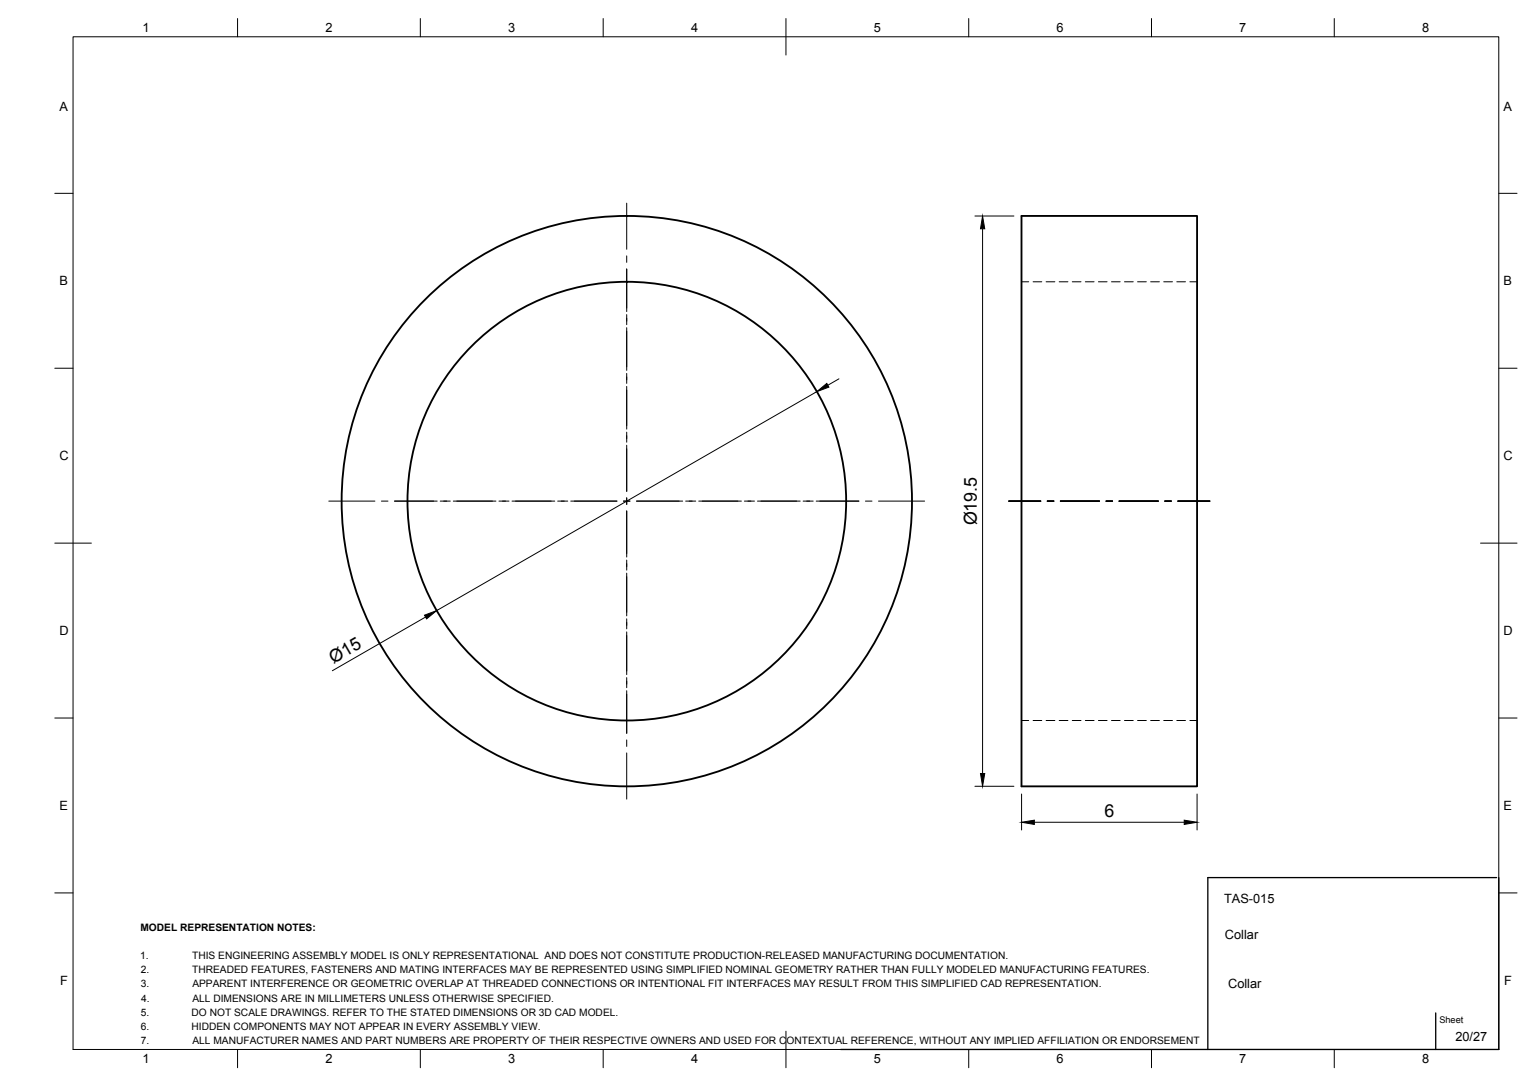
ISO-10303-21;
HEADER;
/* Generated by software containing ST-Developer
 * from STEP Tools, Inc. (www.steptools.com) 
 */

FILE_DESCRIPTION(
/* description */ ('STEP AP214'),
/* implementation_level */ '2;1');

FILE_NAME(
/* name */ 'Collar.step',
/* time_stamp */ '2026-11-15T14:49:54-08:00',
/* author */ (''),
/* organization */ (''),
/* preprocessor_version */ 'ST-DEVELOPER v20.2',
/* originating_system */ 'Autodesk Translation Framework v15.17.0.0',
/* authorisation */ '');

FILE_SCHEMA (('AUTOMOTIVE_DESIGN { 1 0 10303 214 3 1 1 }'));
ENDSEC;

DATA;
#10=MECHANICAL_DESIGN_GEOMETRIC_PRESENTATION_REPRESENTATION('',(#1113),#66721);
#1051=SHAPE_REPRESENTATION_RELATIONSHIP('SRR','None',#66912,#1082);
#1082=ADVANCED_BREP_SHAPE_REPRESENTATION('',(#1148),#66703);
#1113=STYLED_ITEM('',(#67095),#1148);
#1148=MANIFOLD_SOLID_BREP('Body1',#25679);
#1379=FACE_BOUND('',#4754,.T.);
#1380=FACE_BOUND('',#4756,.T.);
#2002=PLANE('',#27675);
#2003=PLANE('',#27676);
#3098=FACE_OUTER_BOUND('',#4751,.T.);
#3099=FACE_OUTER_BOUND('',#4752,.T.);
#3100=FACE_OUTER_BOUND('',#4753,.T.);
#3101=FACE_OUTER_BOUND('',#4755,.T.);
#4751=EDGE_LOOP('',(#20964,#20965,#20966,#20967));
#4752=EDGE_LOOP('',(#20968,#20969,#20970,#20971));
#4753=EDGE_LOOP('',(#20972));
#4754=EDGE_LOOP('',(#20973));
#4755=EDGE_LOOP('',(#20974));
#4756=EDGE_LOOP('',(#20975));
#6854=LINE('',#41115,#8843);
#6855=LINE('',#41121,#8844);
#8843=VECTOR('',#33387,9.75);
#8844=VECTOR('',#33394,7.5);
#10147=CIRCLE('',#27670,9.75);
#10148=CIRCLE('',#27671,9.75);
#10149=CIRCLE('',#27673,7.5);
#10150=CIRCLE('',#27674,7.5);
#12083=VERTEX_POINT('',#41112);
#12084=VERTEX_POINT('',#41114);
#12085=VERTEX_POINT('',#41118);
#12086=VERTEX_POINT('',#41120);
#15175=EDGE_CURVE('',#12083,#12083,#10147,.T.);
#15176=EDGE_CURVE('',#12083,#12084,#6854,.T.);
#15177=EDGE_CURVE('',#12084,#12084,#10148,.T.);
#15178=EDGE_CURVE('',#12085,#12085,#10149,.T.);
#15179=EDGE_CURVE('',#12085,#12086,#6855,.T.);
#15180=EDGE_CURVE('',#12086,#12086,#10150,.T.);
#20964=ORIENTED_EDGE('',*,*,#15175,.F.);
#20965=ORIENTED_EDGE('',*,*,#15176,.T.);
#20966=ORIENTED_EDGE('',*,*,#15177,.T.);
#20967=ORIENTED_EDGE('',*,*,#15176,.F.);
#20968=ORIENTED_EDGE('',*,*,#15178,.F.);
#20969=ORIENTED_EDGE('',*,*,#15179,.T.);
#20970=ORIENTED_EDGE('',*,*,#15180,.T.);
#20971=ORIENTED_EDGE('',*,*,#15179,.F.);
#20972=ORIENTED_EDGE('',*,*,#15175,.T.);
#20973=ORIENTED_EDGE('',*,*,#15180,.F.);
#20974=ORIENTED_EDGE('',*,*,#15177,.F.);
#20975=ORIENTED_EDGE('',*,*,#15178,.T.);
#24087=CYLINDRICAL_SURFACE('',#27669,9.75);
#24088=CYLINDRICAL_SURFACE('',#27672,7.5);
#25051=ADVANCED_FACE('',(#3098),#24087,.T.);
#25052=ADVANCED_FACE('',(#3099),#24088,.F.);
#25053=ADVANCED_FACE('',(#3100,#1379),#2002,.F.);
#25054=ADVANCED_FACE('',(#3101,#1380),#2003,.F.);
#25679=CLOSED_SHELL('',(#25051,#25052,#25053,#25054));
#27668=AXIS2_PLACEMENT_3D('',#41110,#33381,#33382);
#27669=AXIS2_PLACEMENT_3D('',#41111,#33383,#33384);
#27670=AXIS2_PLACEMENT_3D('',#41113,#33385,#33386);
#27671=AXIS2_PLACEMENT_3D('',#41116,#33388,#33389);
#27672=AXIS2_PLACEMENT_3D('',#41117,#33390,#33391);
#27673=AXIS2_PLACEMENT_3D('',#41119,#33392,#33393);
#27674=AXIS2_PLACEMENT_3D('',#41122,#33395,#33396);
#27675=AXIS2_PLACEMENT_3D('',#41123,#33397,#33398);
#27676=AXIS2_PLACEMENT_3D('',#41124,#33399,#33400);
#33381=DIRECTION('axis',(0.,0.,1.));
#33382=DIRECTION('refdir',(1.,0.,0.));
#33383=DIRECTION('center_axis',(-1.,0.,0.));
#33384=DIRECTION('ref_axis',(0.,0.,1.));
#33385=DIRECTION('center_axis',(-1.,0.,0.));
#33386=DIRECTION('ref_axis',(0.,0.,1.));
#33387=DIRECTION('',(1.,0.,0.));
#33388=DIRECTION('center_axis',(-1.,0.,0.));
#33389=DIRECTION('ref_axis',(0.,0.,1.));
#33390=DIRECTION('center_axis',(-1.,0.,0.));
#33391=DIRECTION('ref_axis',(0.,0.,1.));
#33392=DIRECTION('center_axis',(-1.,0.,0.));
#33393=DIRECTION('ref_axis',(0.,0.,1.));
#33394=DIRECTION('',(-1.,0.,0.));
#33395=DIRECTION('center_axis',(-1.,0.,0.));
#33396=DIRECTION('ref_axis',(0.,0.,1.));
#33397=DIRECTION('center_axis',(1.,0.,0.));
#33398=DIRECTION('ref_axis',(0.,0.,-1.));
#33399=DIRECTION('center_axis',(-1.,0.,0.));
#33400=DIRECTION('ref_axis',(0.,0.,1.));
#41110=CARTESIAN_POINT('',(0.,0.,0.));
#41111=CARTESIAN_POINT('Origin',(-0.25,0.,0.));
#41112=CARTESIAN_POINT('',(-3.12250225675825E-16,-1.19403062916867E-15,
-9.75));
#41113=CARTESIAN_POINT('Origin',(-3.25260651745651E-16,0.,0.));
#41114=CARTESIAN_POINT('',(6.,-1.19403062916867E-15,-9.75));
#41115=CARTESIAN_POINT('',(-0.25,-1.19403062916867E-15,-9.75));
#41116=CARTESIAN_POINT('Origin',(6.,0.,0.));
#41117=CARTESIAN_POINT('Origin',(-0.25,0.,0.));
#41118=CARTESIAN_POINT('',(6.,-9.18485099360515E-16,-7.5));
#41119=CARTESIAN_POINT('Origin',(6.,0.,0.));
#41120=CARTESIAN_POINT('',(0.,-9.18485099360515E-16,-7.5));
#41121=CARTESIAN_POINT('',(-0.25,-9.18485099360515E-16,-7.5));
#41122=CARTESIAN_POINT('Origin',(0.,0.,0.));
#41123=CARTESIAN_POINT('Origin',(-1.53080849893419E-16,9.75,0.));
#41124=CARTESIAN_POINT('Origin',(6.,7.5,0.));
#66662=UNCERTAINTY_MEASURE_WITH_UNIT(LENGTH_MEASURE(0.01),#66722,
'DISTANCE_ACCURACY_VALUE',
'Maximum model space distance between geometric entities at asserted c
onnectivities');
#66680=UNCERTAINTY_MEASURE_WITH_UNIT(LENGTH_MEASURE(0.01),#66722,
'DISTANCE_ACCURACY_VALUE',
'Maximum model space distance between geometric entities at asserted c
onnectivities');
#66703=(
GEOMETRIC_REPRESENTATION_CONTEXT(3)
GLOBAL_UNCERTAINTY_ASSIGNED_CONTEXT((#66662))
GLOBAL_UNIT_ASSIGNED_CONTEXT((#66722,#66724,#66725))
REPRESENTATION_CONTEXT('','3D')
);
#66721=(
GEOMETRIC_REPRESENTATION_CONTEXT(3)
GLOBAL_UNCERTAINTY_ASSIGNED_CONTEXT((#66680))
GLOBAL_UNIT_ASSIGNED_CONTEXT((#66722,#66724,#66725))
REPRESENTATION_CONTEXT('','3D')
);
#66722=(
LENGTH_UNIT()
NAMED_UNIT(*)
SI_UNIT(.MILLI.,.METRE.)
);
#66724=(
NAMED_UNIT(*)
PLANE_ANGLE_UNIT()
SI_UNIT($,.RADIAN.)
);
#66725=(
NAMED_UNIT(*)
SI_UNIT($,.STERADIAN.)
SOLID_ANGLE_UNIT()
);
#66748=SHAPE_DEFINITION_REPRESENTATION(#66804,#66912);
#66804=PRODUCT_DEFINITION_SHAPE('',$,#66953);
#66912=SHAPE_REPRESENTATION('',(#27668),#66703);
#66930=PRODUCT_DEFINITION_CONTEXT('part definition',#67052,'design');
#66953=PRODUCT_DEFINITION('Collar','Collar',#66993,#66930);
#66993=PRODUCT_DEFINITION_FORMATION('',$,#67076);
#67052=APPLICATION_CONTEXT(
'Core Data for Automotive Mechanical Design Process');
#67053=PRODUCT_CONTEXT('part definition',#67052,'mechanical');
#67076=PRODUCT('Collar','Collar',$,(#67053));
#67095=PRESENTATION_STYLE_ASSIGNMENT((#67097));
#67097=SURFACE_STYLE_USAGE(.BOTH.,#67099);
#67099=SURFACE_SIDE_STYLE('',(#67101));
#67101=SURFACE_STYLE_FILL_AREA(#67103);
#67103=FILL_AREA_STYLE('Opaque(202,209,238)',(#67105));
#67105=FILL_AREA_STYLE_COLOUR('Opaque(202,209,238)',#67107);
#67107=COLOUR_RGB('Opaque(202,209,238)',0.792156862745098,0.819607843137255,
0.933333333333333);
ENDSEC;
END-ISO-10303-21;
